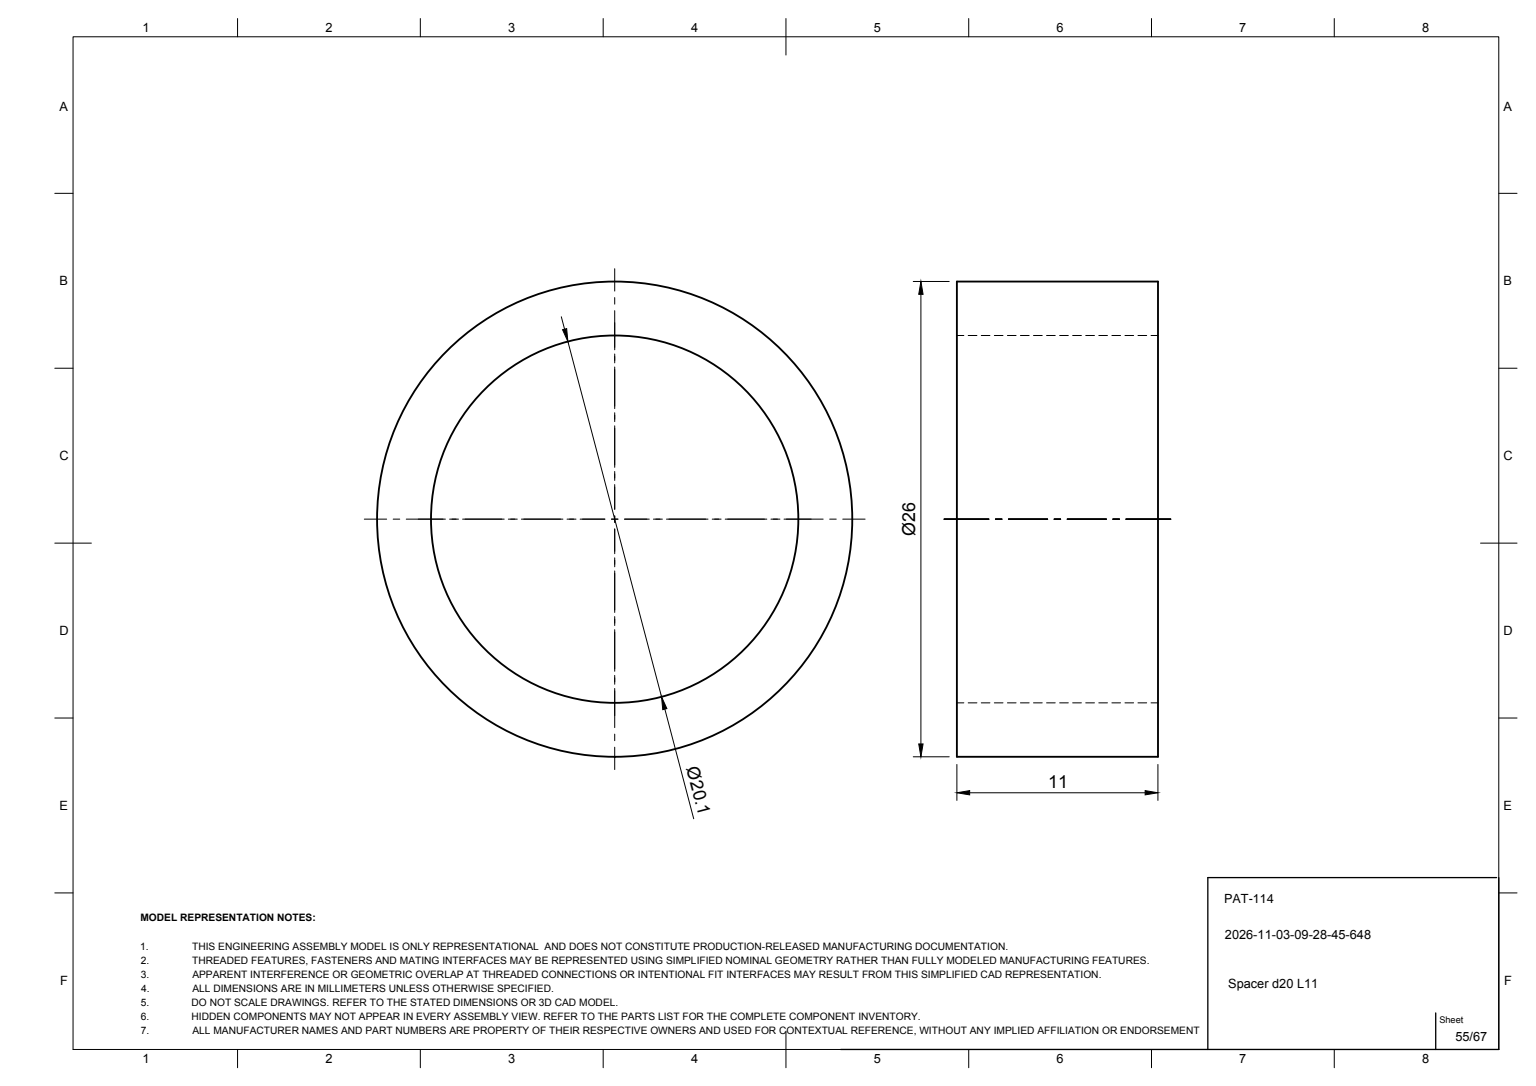
ISO-10303-21;
HEADER;
/* Generated by software containing ST-Developer
 * from STEP Tools, Inc. (www.steptools.com) 
 */

FILE_DESCRIPTION(
/* description */ ('Two-stage gear reducer in split housing'),
/* implementation_level */ '2;1');

FILE_NAME(
/* name */ 'Spacer d20 L11.step',
/* time_stamp */ '2026-10-28T03:22:31-07:00',
/* author */ (''),
/* organization */ (''),
/* preprocessor_version */ 'ST-DEVELOPER v20.2',
/* originating_system */ 'Autodesk Translation Framework v15.17.0.0',
/* authorisation */ '');

FILE_SCHEMA (('AUTOMOTIVE_DESIGN { 1 0 10303 214 3 1 1 }'));
ENDSEC;

DATA;
#10=MECHANICAL_DESIGN_GEOMETRIC_PRESENTATION_REPRESENTATION('',(#1293),#73366);
#1166=SHAPE_REPRESENTATION_RELATIONSHIP('SRR','None',#73657,#1222);
#1222=ADVANCED_BREP_SHAPE_REPRESENTATION('',(#1362),#73353);
#1293=STYLED_ITEM('',(#73974),#1362);
#1362=MANIFOLD_SOLID_BREP('Body1',#16183);
#1576=FACE_BOUND('',#3713,.T.);
#1577=FACE_BOUND('',#3715,.T.);
#1886=PLANE('',#18042);
#1887=PLANE('',#18043);
#2595=FACE_OUTER_BOUND('',#3710,.T.);
#2596=FACE_OUTER_BOUND('',#3711,.T.);
#2597=FACE_OUTER_BOUND('',#3712,.T.);
#2598=FACE_OUTER_BOUND('',#3714,.T.);
#3710=EDGE_LOOP('',(#13155,#13156,#13157,#13158));
#3711=EDGE_LOOP('',(#13159,#13160,#13161,#13162));
#3712=EDGE_LOOP('',(#13163));
#3713=EDGE_LOOP('',(#13164));
#3714=EDGE_LOOP('',(#13165));
#3715=EDGE_LOOP('',(#13166));
#4702=LINE('',#37651,#5726);
#4703=LINE('',#37657,#5727);
#5726=VECTOR('',#21556,1.005);
#5727=VECTOR('',#21563,1.3);
#6654=CIRCLE('',#18037,1.005);
#6655=CIRCLE('',#18038,1.005);
#6656=CIRCLE('',#18040,1.3);
#6657=CIRCLE('',#18041,1.3);
#7723=VERTEX_POINT('',#37648);
#7724=VERTEX_POINT('',#37650);
#7725=VERTEX_POINT('',#37654);
#7726=VERTEX_POINT('',#37656);
#9631=EDGE_CURVE('',#7723,#7723,#6654,.T.);
#9632=EDGE_CURVE('',#7723,#7724,#4702,.T.);
#9633=EDGE_CURVE('',#7724,#7724,#6655,.T.);
#9634=EDGE_CURVE('',#7725,#7725,#6656,.T.);
#9635=EDGE_CURVE('',#7725,#7726,#4703,.T.);
#9636=EDGE_CURVE('',#7726,#7726,#6657,.T.);
#13155=ORIENTED_EDGE('',*,*,#9631,.F.);
#13156=ORIENTED_EDGE('',*,*,#9632,.T.);
#13157=ORIENTED_EDGE('',*,*,#9633,.T.);
#13158=ORIENTED_EDGE('',*,*,#9632,.F.);
#13159=ORIENTED_EDGE('',*,*,#9634,.F.);
#13160=ORIENTED_EDGE('',*,*,#9635,.T.);
#13161=ORIENTED_EDGE('',*,*,#9636,.T.);
#13162=ORIENTED_EDGE('',*,*,#9635,.F.);
#13163=ORIENTED_EDGE('',*,*,#9634,.T.);
#13164=ORIENTED_EDGE('',*,*,#9631,.T.);
#13165=ORIENTED_EDGE('',*,*,#9636,.F.);
#13166=ORIENTED_EDGE('',*,*,#9633,.F.);
#15127=CYLINDRICAL_SURFACE('',#18036,1.005);
#15128=CYLINDRICAL_SURFACE('',#18039,1.3);
#15802=ADVANCED_FACE('',(#2595),#15127,.F.);
#15803=ADVANCED_FACE('',(#2596),#15128,.T.);
#15804=ADVANCED_FACE('',(#2597,#1576),#1886,.T.);
#15805=ADVANCED_FACE('',(#2598,#1577),#1887,.F.);
#16183=CLOSED_SHELL('',(#15802,#15803,#15804,#15805));
#18035=AXIS2_PLACEMENT_3D('',#37646,#21550,#21551);
#18036=AXIS2_PLACEMENT_3D('',#37647,#21552,#21553);
#18037=AXIS2_PLACEMENT_3D('',#37649,#21554,#21555);
#18038=AXIS2_PLACEMENT_3D('',#37652,#21557,#21558);
#18039=AXIS2_PLACEMENT_3D('',#37653,#21559,#21560);
#18040=AXIS2_PLACEMENT_3D('',#37655,#21561,#21562);
#18041=AXIS2_PLACEMENT_3D('',#37658,#21564,#21565);
#18042=AXIS2_PLACEMENT_3D('',#37659,#21566,#21567);
#18043=AXIS2_PLACEMENT_3D('',#37660,#21568,#21569);
#21550=DIRECTION('axis',(0.,0.,1.));
#21551=DIRECTION('refdir',(1.,0.,0.));
#21552=DIRECTION('center_axis',(0.,1.,0.));
#21553=DIRECTION('ref_axis',(1.,0.,0.));
#21554=DIRECTION('center_axis',(0.,-1.,0.));
#21555=DIRECTION('ref_axis',(1.,0.,0.));
#21556=DIRECTION('',(0.,-1.,0.));
#21557=DIRECTION('center_axis',(0.,-1.,0.));
#21558=DIRECTION('ref_axis',(1.,0.,0.));
#21559=DIRECTION('center_axis',(0.,1.,0.));
#21560=DIRECTION('ref_axis',(1.,0.,0.));
#21561=DIRECTION('center_axis',(0.,1.,0.));
#21562=DIRECTION('ref_axis',(1.,0.,0.));
#21563=DIRECTION('',(0.,-1.,0.));
#21564=DIRECTION('center_axis',(0.,1.,0.));
#21565=DIRECTION('ref_axis',(1.,0.,0.));
#21566=DIRECTION('center_axis',(0.,1.,0.));
#21567=DIRECTION('ref_axis',(1.,0.,0.));
#21568=DIRECTION('center_axis',(0.,1.,0.));
#21569=DIRECTION('ref_axis',(1.,0.,0.));
#37646=CARTESIAN_POINT('',(0.,0.,0.));
#37647=CARTESIAN_POINT('Origin',(6.,4.2,10.));
#37648=CARTESIAN_POINT('',(4.995,5.3,10.));
#37649=CARTESIAN_POINT('Origin',(6.,5.3,10.));
#37650=CARTESIAN_POINT('',(4.995,4.2,10.));
#37651=CARTESIAN_POINT('',(4.995,4.2,10.));
#37652=CARTESIAN_POINT('Origin',(6.,4.2,10.));
#37653=CARTESIAN_POINT('Origin',(6.,4.2,10.));
#37654=CARTESIAN_POINT('',(4.7,5.3,10.));
#37655=CARTESIAN_POINT('Origin',(6.,5.3,10.));
#37656=CARTESIAN_POINT('',(4.7,4.2,10.));
#37657=CARTESIAN_POINT('',(4.7,4.2,10.));
#37658=CARTESIAN_POINT('Origin',(6.,4.2,10.));
#37659=CARTESIAN_POINT('Origin',(6.,5.3,10.));
#37660=CARTESIAN_POINT('Origin',(6.,4.2,10.));
#73289=UNCERTAINTY_MEASURE_WITH_UNIT(LENGTH_MEASURE(0.001),#73367,
'DISTANCE_ACCURACY_VALUE',
'Maximum model space distance between geometric entities at asserted c
onnectivities');
#73302=UNCERTAINTY_MEASURE_WITH_UNIT(LENGTH_MEASURE(0.001),#73367,
'DISTANCE_ACCURACY_VALUE',
'Maximum model space distance between geometric entities at asserted c
onnectivities');
#73353=(
GEOMETRIC_REPRESENTATION_CONTEXT(3)
GLOBAL_UNCERTAINTY_ASSIGNED_CONTEXT((#73289))
GLOBAL_UNIT_ASSIGNED_CONTEXT((#73367,#73369,#73370))
REPRESENTATION_CONTEXT('','3D')
);
#73366=(
GEOMETRIC_REPRESENTATION_CONTEXT(3)
GLOBAL_UNCERTAINTY_ASSIGNED_CONTEXT((#73302))
GLOBAL_UNIT_ASSIGNED_CONTEXT((#73367,#73369,#73370))
REPRESENTATION_CONTEXT('','3D')
);
#73367=(
LENGTH_UNIT()
NAMED_UNIT(*)
SI_UNIT(.CENTI.,.METRE.)
);
#73369=(
NAMED_UNIT(*)
PLANE_ANGLE_UNIT()
SI_UNIT($,.RADIAN.)
);
#73370=(
NAMED_UNIT(*)
SI_UNIT($,.STERADIAN.)
SOLID_ANGLE_UNIT()
);
#73421=SHAPE_DEFINITION_REPRESENTATION(#73554,#73657);
#73554=PRODUCT_DEFINITION_SHAPE('',$,#73721);
#73657=SHAPE_REPRESENTATION('',(#18035),#73353);
#73670=PRODUCT_DEFINITION_CONTEXT('part definition',#73861,'design');
#73721=PRODUCT_DEFINITION('Spacer d20 L11','Spacer d20 L11',#73784,#73670);
#73784=PRODUCT_DEFINITION_FORMATION('',$,#73913);
#73861=APPLICATION_CONTEXT(
'Core Data for Automotive Mechanical Design Process');
#73862=PRODUCT_CONTEXT('part definition',#73861,'mechanical');
#73913=PRODUCT('Spacer d20 L11','Spacer d20 L11','Spacer d20 L11',(#73862));
#73968=COLOUR_RGB('Light Blue',0.38,0.62,0.78);
#73969=FILL_AREA_STYLE_COLOUR('',#73968);
#73970=FILL_AREA_STYLE('',(#73969));
#73971=SURFACE_STYLE_FILL_AREA(#73970);
#73972=SURFACE_SIDE_STYLE('',(#73971));
#73973=SURFACE_STYLE_USAGE(.BOTH.,#73972);
#73974=PRESENTATION_STYLE_ASSIGNMENT((#73973));
ENDSEC;
END-ISO-10303-21;
